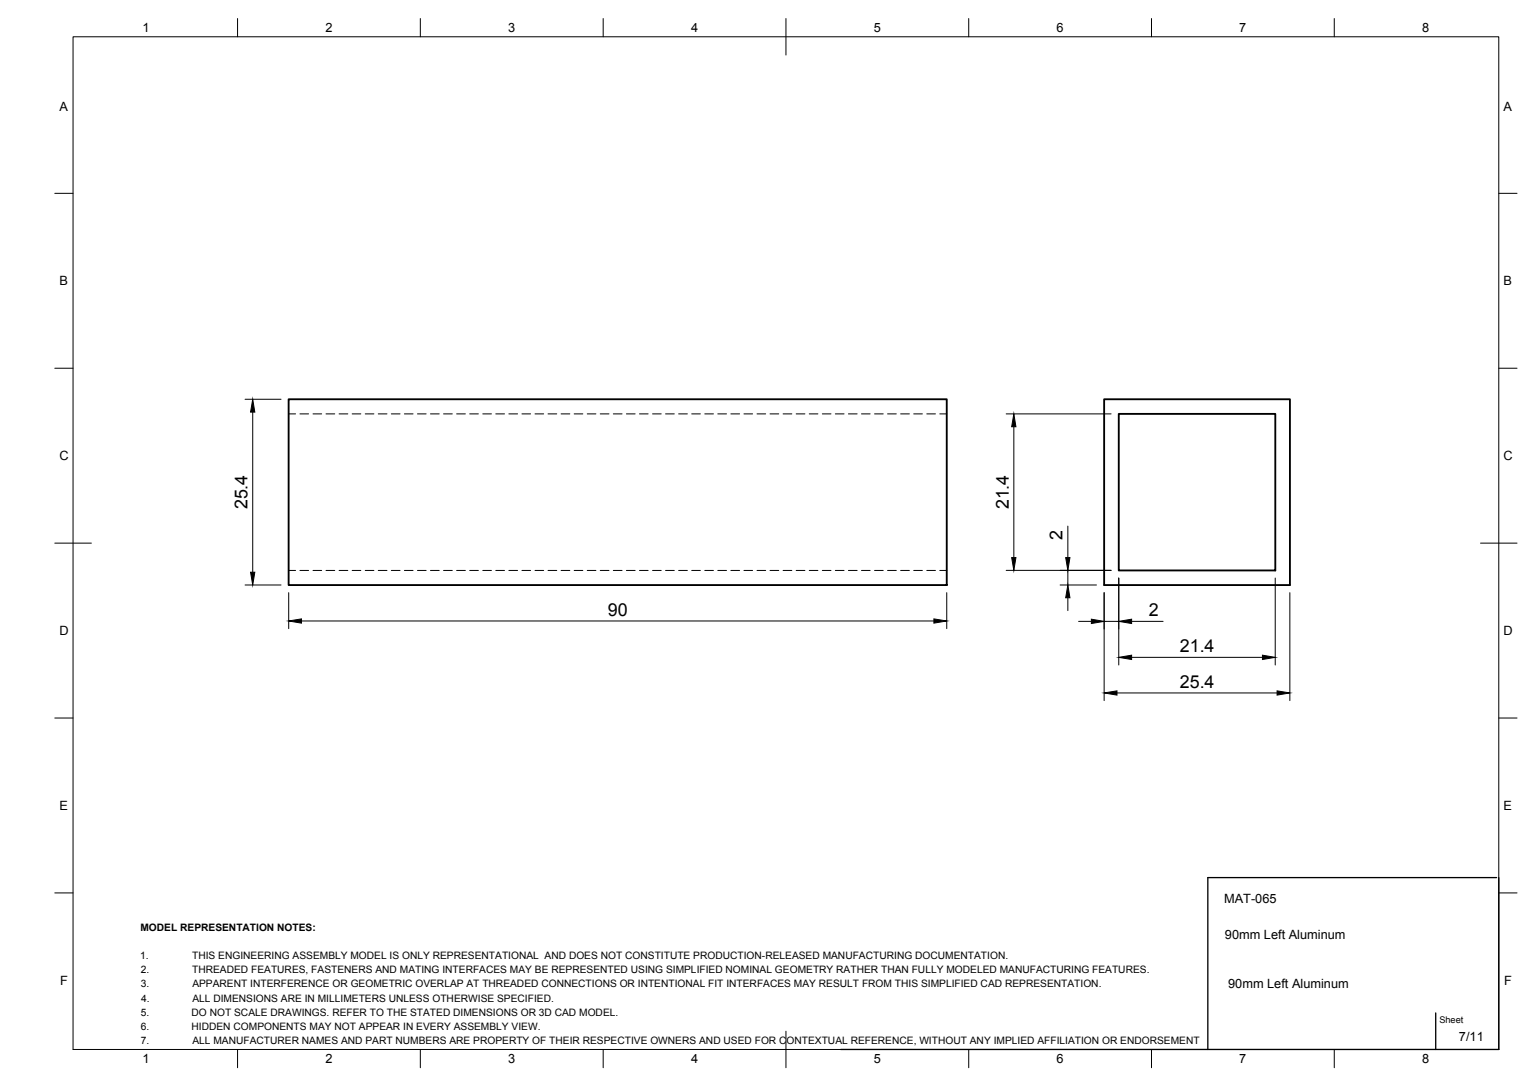
ISO-10303-21;
HEADER;
/* Generated by software containing ST-Developer
 * from STEP Tools, Inc. (www.steptools.com) 
 */

FILE_DESCRIPTION(
/* description */ (
'CAx-IF Rec.Pracs.---Representation and Presentation of Product Manufa
cturing Information (PMI)---4.0---2014-10-13'),
/* implementation_level */ '2;1');

FILE_NAME(
/* name */ '90mm Left Aluminum.step',
/* time_stamp */ '2026-11-15T23:28:27-08:00',
/* author */ (''),
/* organization */ (''),
/* preprocessor_version */ 'ST-DEVELOPER v20.2',
/* originating_system */ 'Autodesk Translation Framework v15.17.0.0',
/* authorisation */ '');

FILE_SCHEMA (('AUTOMOTIVE_DESIGN { 1 0 10303 214 3 1 1 }'));
ENDSEC;

DATA;
#10=MECHANICAL_DESIGN_GEOMETRIC_PRESENTATION_REPRESENTATION('',(#190),#7756);
#172=SHAPE_REPRESENTATION_RELATIONSHIP('SRR','None',#7820,#181);
#181=ADVANCED_BREP_SHAPE_REPRESENTATION('',(#199),#7748);
#190=STYLED_ITEM('',(#7874),#199);
#199=MANIFOLD_SOLID_BREP('Body1',#4627);
#390=FACE_BOUND('',#721,.T.);
#391=FACE_BOUND('',#723,.T.);
#467=FACE_OUTER_BOUND('',#712,.T.);
#468=FACE_OUTER_BOUND('',#713,.T.);
#469=FACE_OUTER_BOUND('',#714,.T.);
#470=FACE_OUTER_BOUND('',#715,.T.);
#471=FACE_OUTER_BOUND('',#716,.T.);
#472=FACE_OUTER_BOUND('',#717,.T.);
#473=FACE_OUTER_BOUND('',#718,.T.);
#474=FACE_OUTER_BOUND('',#719,.T.);
#475=FACE_OUTER_BOUND('',#720,.T.);
#476=FACE_OUTER_BOUND('',#722,.T.);
#712=EDGE_LOOP('',(#3071,#3072,#3073,#3074));
#713=EDGE_LOOP('',(#3075,#3076,#3077,#3078));
#714=EDGE_LOOP('',(#3079,#3080,#3081,#3082));
#715=EDGE_LOOP('',(#3083,#3084,#3085,#3086));
#716=EDGE_LOOP('',(#3087,#3088,#3089,#3090));
#717=EDGE_LOOP('',(#3091,#3092,#3093,#3094));
#718=EDGE_LOOP('',(#3095,#3096,#3097,#3098));
#719=EDGE_LOOP('',(#3099,#3100,#3101,#3102));
#720=EDGE_LOOP('',(#3103,#3104,#3105,#3106));
#721=EDGE_LOOP('',(#3107,#3108,#3109,#3110));
#722=EDGE_LOOP('',(#3111,#3112,#3113,#3114));
#723=EDGE_LOOP('',(#3115,#3116,#3117,#3118));
#1021=LINE('',#6505,#1514);
#1022=LINE('',#6507,#1515);
#1023=LINE('',#6509,#1516);
#1024=LINE('',#6510,#1517);
#1025=LINE('',#6513,#1518);
#1026=LINE('',#6515,#1519);
#1027=LINE('',#6516,#1520);
#1028=LINE('',#6519,#1521);
#1029=LINE('',#6521,#1522);
#1030=LINE('',#6522,#1523);
#1031=LINE('',#6526,#1524);
#1032=LINE('',#6528,#1525);
#1033=LINE('',#6530,#1526);
#1034=LINE('',#6531,#1527);
#1035=LINE('',#6534,#1528);
#1036=LINE('',#6536,#1529);
#1037=LINE('',#6537,#1530);
#1038=LINE('',#6540,#1531);
#1039=LINE('',#6542,#1532);
#1040=LINE('',#6543,#1533);
#1041=LINE('',#6545,#1534);
#1042=LINE('',#6546,#1535);
#1043=LINE('',#6548,#1536);
#1044=LINE('',#6549,#1537);
#1514=VECTOR('',#5219,1.);
#1515=VECTOR('',#5220,1.);
#1516=VECTOR('',#5221,1.);
#1517=VECTOR('',#5222,1.);
#1518=VECTOR('',#5225,1.);
#1519=VECTOR('',#5226,1.);
#1520=VECTOR('',#5227,1.);
#1521=VECTOR('',#5230,1.);
#1522=VECTOR('',#5231,1.);
#1523=VECTOR('',#5232,1.);
#1524=VECTOR('',#5235,1.);
#1525=VECTOR('',#5236,1.);
#1526=VECTOR('',#5237,1.);
#1527=VECTOR('',#5238,1.);
#1528=VECTOR('',#5241,1.);
#1529=VECTOR('',#5242,1.);
#1530=VECTOR('',#5243,1.);
#1531=VECTOR('',#5246,1.);
#1532=VECTOR('',#5247,1.);
#1533=VECTOR('',#5248,1.);
#1534=VECTOR('',#5251,1.);
#1535=VECTOR('',#5252,1.);
#1536=VECTOR('',#5255,1.);
#1537=VECTOR('',#5256,1.);
#2004=VERTEX_POINT('',#6503);
#2005=VERTEX_POINT('',#6504);
#2006=VERTEX_POINT('',#6506);
#2007=VERTEX_POINT('',#6508);
#2008=VERTEX_POINT('',#6512);
#2009=VERTEX_POINT('',#6514);
#2010=VERTEX_POINT('',#6518);
#2011=VERTEX_POINT('',#6520);
#2012=VERTEX_POINT('',#6524);
#2013=VERTEX_POINT('',#6525);
#2014=VERTEX_POINT('',#6527);
#2015=VERTEX_POINT('',#6529);
#2016=VERTEX_POINT('',#6533);
#2017=VERTEX_POINT('',#6535);
#2018=VERTEX_POINT('',#6539);
#2019=VERTEX_POINT('',#6541);
#2419=EDGE_CURVE('',#2004,#2005,#1021,.T.);
#2420=EDGE_CURVE('',#2006,#2004,#1022,.T.);
#2421=EDGE_CURVE('',#2006,#2007,#1023,.T.);
#2422=EDGE_CURVE('',#2007,#2005,#1024,.T.);
#2423=EDGE_CURVE('',#2004,#2008,#1025,.T.);
#2424=EDGE_CURVE('',#2009,#2008,#1026,.T.);
#2425=EDGE_CURVE('',#2006,#2009,#1027,.T.);
#2426=EDGE_CURVE('',#2008,#2010,#1028,.T.);
#2427=EDGE_CURVE('',#2011,#2010,#1029,.T.);
#2428=EDGE_CURVE('',#2009,#2011,#1030,.T.);
#2429=EDGE_CURVE('',#2012,#2013,#1031,.T.);
#2430=EDGE_CURVE('',#2014,#2012,#1032,.T.);
#2431=EDGE_CURVE('',#2014,#2015,#1033,.T.);
#2432=EDGE_CURVE('',#2015,#2013,#1034,.T.);
#2433=EDGE_CURVE('',#2012,#2016,#1035,.T.);
#2434=EDGE_CURVE('',#2017,#2016,#1036,.T.);
#2435=EDGE_CURVE('',#2014,#2017,#1037,.T.);
#2436=EDGE_CURVE('',#2016,#2018,#1038,.T.);
#2437=EDGE_CURVE('',#2019,#2018,#1039,.T.);
#2438=EDGE_CURVE('',#2017,#2019,#1040,.T.);
#2439=EDGE_CURVE('',#2013,#2018,#1041,.T.);
#2440=EDGE_CURVE('',#2015,#2019,#1042,.T.);
#2441=EDGE_CURVE('',#2005,#2010,#1043,.T.);
#2442=EDGE_CURVE('',#2007,#2011,#1044,.T.);
#3071=ORIENTED_EDGE('',*,*,#2419,.F.);
#3072=ORIENTED_EDGE('',*,*,#2420,.F.);
#3073=ORIENTED_EDGE('',*,*,#2421,.T.);
#3074=ORIENTED_EDGE('',*,*,#2422,.T.);
#3075=ORIENTED_EDGE('',*,*,#2423,.T.);
#3076=ORIENTED_EDGE('',*,*,#2424,.F.);
#3077=ORIENTED_EDGE('',*,*,#2425,.F.);
#3078=ORIENTED_EDGE('',*,*,#2420,.T.);
#3079=ORIENTED_EDGE('',*,*,#2426,.T.);
#3080=ORIENTED_EDGE('',*,*,#2427,.F.);
#3081=ORIENTED_EDGE('',*,*,#2428,.F.);
#3082=ORIENTED_EDGE('',*,*,#2424,.T.);
#3083=ORIENTED_EDGE('',*,*,#2429,.F.);
#3084=ORIENTED_EDGE('',*,*,#2430,.F.);
#3085=ORIENTED_EDGE('',*,*,#2431,.T.);
#3086=ORIENTED_EDGE('',*,*,#2432,.T.);
#3087=ORIENTED_EDGE('',*,*,#2433,.T.);
#3088=ORIENTED_EDGE('',*,*,#2434,.F.);
#3089=ORIENTED_EDGE('',*,*,#2435,.F.);
#3090=ORIENTED_EDGE('',*,*,#2430,.T.);
#3091=ORIENTED_EDGE('',*,*,#2436,.T.);
#3092=ORIENTED_EDGE('',*,*,#2437,.F.);
#3093=ORIENTED_EDGE('',*,*,#2438,.F.);
#3094=ORIENTED_EDGE('',*,*,#2434,.T.);
#3095=ORIENTED_EDGE('',*,*,#2439,.F.);
#3096=ORIENTED_EDGE('',*,*,#2432,.F.);
#3097=ORIENTED_EDGE('',*,*,#2440,.T.);
#3098=ORIENTED_EDGE('',*,*,#2437,.T.);
#3099=ORIENTED_EDGE('',*,*,#2441,.F.);
#3100=ORIENTED_EDGE('',*,*,#2422,.F.);
#3101=ORIENTED_EDGE('',*,*,#2442,.T.);
#3102=ORIENTED_EDGE('',*,*,#2427,.T.);
#3103=ORIENTED_EDGE('',*,*,#2421,.F.);
#3104=ORIENTED_EDGE('',*,*,#2425,.T.);
#3105=ORIENTED_EDGE('',*,*,#2428,.T.);
#3106=ORIENTED_EDGE('',*,*,#2442,.F.);
#3107=ORIENTED_EDGE('',*,*,#2431,.F.);
#3108=ORIENTED_EDGE('',*,*,#2435,.T.);
#3109=ORIENTED_EDGE('',*,*,#2438,.T.);
#3110=ORIENTED_EDGE('',*,*,#2440,.F.);
#3111=ORIENTED_EDGE('',*,*,#2419,.T.);
#3112=ORIENTED_EDGE('',*,*,#2441,.T.);
#3113=ORIENTED_EDGE('',*,*,#2426,.F.);
#3114=ORIENTED_EDGE('',*,*,#2423,.F.);
#3115=ORIENTED_EDGE('',*,*,#2429,.T.);
#3116=ORIENTED_EDGE('',*,*,#2439,.T.);
#3117=ORIENTED_EDGE('',*,*,#2436,.F.);
#3118=ORIENTED_EDGE('',*,*,#2433,.F.);
#4229=PLANE('',#4763);
#4230=PLANE('',#4764);
#4231=PLANE('',#4765);
#4232=PLANE('',#4766);
#4233=PLANE('',#4767);
#4234=PLANE('',#4768);
#4235=PLANE('',#4769);
#4236=PLANE('',#4770);
#4237=PLANE('',#4771);
#4238=PLANE('',#4772);
#4408=ADVANCED_FACE('',(#467),#4229,.T.);
#4409=ADVANCED_FACE('',(#468),#4230,.F.);
#4410=ADVANCED_FACE('',(#469),#4231,.F.);
#4411=ADVANCED_FACE('',(#470),#4232,.T.);
#4412=ADVANCED_FACE('',(#471),#4233,.F.);
#4413=ADVANCED_FACE('',(#472),#4234,.F.);
#4414=ADVANCED_FACE('',(#473),#4235,.T.);
#4415=ADVANCED_FACE('',(#474),#4236,.T.);
#4416=ADVANCED_FACE('',(#475,#390),#4237,.T.);
#4417=ADVANCED_FACE('',(#476,#391),#4238,.F.);
#4627=CLOSED_SHELL('',(#4408,#4409,#4410,#4411,#4412,#4413,#4414,#4415,
#4416,#4417));
#4762=AXIS2_PLACEMENT_3D('',#6501,#5215,#5216);
#4763=AXIS2_PLACEMENT_3D('',#6502,#5217,#5218);
#4764=AXIS2_PLACEMENT_3D('',#6511,#5223,#5224);
#4765=AXIS2_PLACEMENT_3D('',#6517,#5228,#5229);
#4766=AXIS2_PLACEMENT_3D('',#6523,#5233,#5234);
#4767=AXIS2_PLACEMENT_3D('',#6532,#5239,#5240);
#4768=AXIS2_PLACEMENT_3D('',#6538,#5244,#5245);
#4769=AXIS2_PLACEMENT_3D('',#6544,#5249,#5250);
#4770=AXIS2_PLACEMENT_3D('',#6547,#5253,#5254);
#4771=AXIS2_PLACEMENT_3D('',#6550,#5257,#5258);
#4772=AXIS2_PLACEMENT_3D('',#6551,#5259,#5260);
#5215=DIRECTION('axis',(0.,0.,1.));
#5216=DIRECTION('refdir',(1.,0.,0.));
#5217=DIRECTION('center_axis',(0.,1.,0.));
#5218=DIRECTION('ref_axis',(0.,0.,1.));
#5219=DIRECTION('',(1.,0.,0.));
#5220=DIRECTION('',(0.,0.,-1.));
#5221=DIRECTION('',(1.,0.,0.));
#5222=DIRECTION('',(0.,0.,-1.));
#5223=DIRECTION('center_axis',(1.,0.,0.));
#5224=DIRECTION('ref_axis',(0.,0.,-1.));
#5225=DIRECTION('',(0.,-1.,0.));
#5226=DIRECTION('',(0.,0.,-1.));
#5227=DIRECTION('',(0.,-1.,0.));
#5228=DIRECTION('center_axis',(0.,1.,0.));
#5229=DIRECTION('ref_axis',(0.,0.,1.));
#5230=DIRECTION('',(1.,0.,0.));
#5231=DIRECTION('',(0.,0.,-1.));
#5232=DIRECTION('',(1.,0.,0.));
#5233=DIRECTION('center_axis',(1.,0.,0.));
#5234=DIRECTION('ref_axis',(0.,0.,-1.));
#5235=DIRECTION('',(0.,-1.,0.));
#5236=DIRECTION('',(0.,0.,-1.));
#5237=DIRECTION('',(0.,-1.,0.));
#5238=DIRECTION('',(0.,0.,-1.));
#5239=DIRECTION('center_axis',(0.,1.,0.));
#5240=DIRECTION('ref_axis',(0.,0.,1.));
#5241=DIRECTION('',(1.,0.,0.));
#5242=DIRECTION('',(0.,0.,-1.));
#5243=DIRECTION('',(1.,0.,0.));
#5244=DIRECTION('center_axis',(1.,0.,0.));
#5245=DIRECTION('ref_axis',(0.,0.,-1.));
#5246=DIRECTION('',(0.,-1.,0.));
#5247=DIRECTION('',(0.,0.,-1.));
#5248=DIRECTION('',(0.,-1.,0.));
#5249=DIRECTION('center_axis',(0.,1.,0.));
#5250=DIRECTION('ref_axis',(0.,0.,1.));
#5251=DIRECTION('',(1.,0.,0.));
#5252=DIRECTION('',(1.,0.,0.));
#5253=DIRECTION('center_axis',(1.,0.,0.));
#5254=DIRECTION('ref_axis',(0.,0.,-1.));
#5255=DIRECTION('',(0.,-1.,0.));
#5256=DIRECTION('',(0.,-1.,0.));
#5257=DIRECTION('center_axis',(0.,0.,1.));
#5258=DIRECTION('ref_axis',(1.,0.,0.));
#5259=DIRECTION('center_axis',(0.,0.,1.));
#5260=DIRECTION('ref_axis',(1.,0.,0.));
#6501=CARTESIAN_POINT('',(0.,0.,0.));
#6502=CARTESIAN_POINT('Origin',(0.0208455896936357,0.0585086531437975,0.09));
#6503=CARTESIAN_POINT('',(0.0081455896936357,0.0585086531437975,0.));
#6504=CARTESIAN_POINT('',(0.0335455896936357,0.0585086531437975,0.));
#6505=CARTESIAN_POINT('',(0.0208455896936357,0.0585086531437975,0.));
#6506=CARTESIAN_POINT('',(0.0081455896936357,0.0585086531437975,0.09));
#6507=CARTESIAN_POINT('',(0.0081455896936357,0.0585086531437975,0.09));
#6508=CARTESIAN_POINT('',(0.0335455896936357,0.0585086531437975,0.09));
#6509=CARTESIAN_POINT('',(0.0208455896936357,0.0585086531437975,0.09));
#6510=CARTESIAN_POINT('',(0.0335455896936357,0.0585086531437975,0.09));
#6511=CARTESIAN_POINT('Origin',(0.0081455896936357,0.0458086531437975,0.09));
#6512=CARTESIAN_POINT('',(0.0081455896936357,0.0331086531437976,0.));
#6513=CARTESIAN_POINT('',(0.0081455896936357,0.0458086531437975,0.));
#6514=CARTESIAN_POINT('',(0.0081455896936357,0.0331086531437976,0.09));
#6515=CARTESIAN_POINT('',(0.0081455896936357,0.0331086531437976,0.09));
#6516=CARTESIAN_POINT('',(0.0081455896936357,0.0458086531437975,0.09));
#6517=CARTESIAN_POINT('Origin',(0.0208455896936357,0.0331086531437976,0.09));
#6518=CARTESIAN_POINT('',(0.0335455896936357,0.0331086531437976,0.));
#6519=CARTESIAN_POINT('',(0.0208455896936357,0.0331086531437976,0.));
#6520=CARTESIAN_POINT('',(0.0335455896936357,0.0331086531437976,0.09));
#6521=CARTESIAN_POINT('',(0.0335455896936357,0.0331086531437976,0.09));
#6522=CARTESIAN_POINT('',(0.0208455896936357,0.0331086531437976,0.09));
#6523=CARTESIAN_POINT('Origin',(0.0101455896936357,0.0458086531437976,0.09));
#6524=CARTESIAN_POINT('',(0.0101455896936357,0.0565086531437975,0.));
#6525=CARTESIAN_POINT('',(0.0101455896936357,0.0351086531437975,0.));
#6526=CARTESIAN_POINT('',(0.0101455896936357,0.0458086531437976,0.));
#6527=CARTESIAN_POINT('',(0.0101455896936357,0.0565086531437975,0.09));
#6528=CARTESIAN_POINT('',(0.0101455896936357,0.0565086531437975,0.09));
#6529=CARTESIAN_POINT('',(0.0101455896936357,0.0351086531437975,0.09));
#6530=CARTESIAN_POINT('',(0.0101455896936357,0.0458086531437976,0.09));
#6531=CARTESIAN_POINT('',(0.0101455896936357,0.0351086531437975,0.09));
#6532=CARTESIAN_POINT('Origin',(0.0208455896936357,0.0565086531437975,0.09));
#6533=CARTESIAN_POINT('',(0.0315455896936357,0.0565086531437975,0.));
#6534=CARTESIAN_POINT('',(0.0208455896936357,0.0565086531437975,0.));
#6535=CARTESIAN_POINT('',(0.0315455896936357,0.0565086531437975,0.09));
#6536=CARTESIAN_POINT('',(0.0315455896936357,0.0565086531437975,0.09));
#6537=CARTESIAN_POINT('',(0.0208455896936357,0.0565086531437975,0.09));
#6538=CARTESIAN_POINT('Origin',(0.0315455896936357,0.0458086531437976,0.09));
#6539=CARTESIAN_POINT('',(0.0315455896936357,0.0351086531437975,0.));
#6540=CARTESIAN_POINT('',(0.0315455896936357,0.0458086531437976,0.));
#6541=CARTESIAN_POINT('',(0.0315455896936357,0.0351086531437975,0.09));
#6542=CARTESIAN_POINT('',(0.0315455896936357,0.0351086531437975,0.09));
#6543=CARTESIAN_POINT('',(0.0315455896936357,0.0458086531437976,0.09));
#6544=CARTESIAN_POINT('Origin',(0.0208455896936357,0.0351086531437975,0.09));
#6545=CARTESIAN_POINT('',(0.0208455896936357,0.0351086531437975,0.));
#6546=CARTESIAN_POINT('',(0.0208455896936357,0.0351086531437975,0.09));
#6547=CARTESIAN_POINT('Origin',(0.0335455896936357,0.0458086531437975,0.09));
#6548=CARTESIAN_POINT('',(0.0335455896936357,0.0458086531437975,0.));
#6549=CARTESIAN_POINT('',(0.0335455896936357,0.0458086531437975,0.09));
#6550=CARTESIAN_POINT('Origin',(0.0208455896936357,0.0458086531437975,0.09));
#6551=CARTESIAN_POINT('Origin',(0.0208455896936357,0.0458086531437975,0.));
#7737=UNCERTAINTY_MEASURE_WITH_UNIT(LENGTH_MEASURE(1.E-5),#7757,
'DISTANCE_ACCURACY_VALUE',
'Maximum model space distance between geometric entities at asserted c
onnectivities');
#7745=UNCERTAINTY_MEASURE_WITH_UNIT(LENGTH_MEASURE(1.E-5),#7757,
'DISTANCE_ACCURACY_VALUE',
'Maximum model space distance between geometric entities at asserted c
onnectivities');
#7748=(
GEOMETRIC_REPRESENTATION_CONTEXT(3)
GLOBAL_UNCERTAINTY_ASSIGNED_CONTEXT((#7737))
GLOBAL_UNIT_ASSIGNED_CONTEXT((#7757,#7758,#7759))
REPRESENTATION_CONTEXT('','3D')
);
#7756=(
GEOMETRIC_REPRESENTATION_CONTEXT(3)
GLOBAL_UNCERTAINTY_ASSIGNED_CONTEXT((#7745))
GLOBAL_UNIT_ASSIGNED_CONTEXT((#7757,#7758,#7759))
REPRESENTATION_CONTEXT('','3D')
);
#7757=(
LENGTH_UNIT()
NAMED_UNIT(*)
SI_UNIT($,.METRE.)
);
#7758=(
NAMED_UNIT(*)
PLANE_ANGLE_UNIT()
SI_UNIT($,.RADIAN.)
);
#7759=(
NAMED_UNIT(*)
SI_UNIT($,.STERADIAN.)
SOLID_ANGLE_UNIT()
);
#7762=SHAPE_DEFINITION_REPRESENTATION(#7772,#7820);
#7772=PRODUCT_DEFINITION_SHAPE('',$,#7831);
#7820=SHAPE_REPRESENTATION('',(#4762),#7748);
#7828=PRODUCT_DEFINITION_CONTEXT('part definition',#7860,'design');
#7831=PRODUCT_DEFINITION('90mm Left Aluminum','90mm Left Aluminum',#7841,
#7828);
#7841=PRODUCT_DEFINITION_FORMATION('',$,#7864);
#7860=APPLICATION_CONTEXT(
'Core Data for Automotive Mechanical Design Process');
#7861=PRODUCT_CONTEXT('part definition',#7860,'mechanical');
#7864=PRODUCT('90mm Left Aluminum','90mm Left Aluminum',
'LEGAL AND USAGE DISCLAIMER: this Data/Model is provided \X2\201C\X0\A
S IS\X2\201D\X0\ for informational and representational only. It is a 
geometric approximation and is NOT engineered, certified, or guarantee
d for dimensional accuracy, exact tolerances, or production-level prec
ision. Vendor disclaims all implied warranties including fitness for a
 particular purpose. DO NOT USE FOR DIRECT PHYSICAL MANUFACTURING, AUT
OMATED PRODUCTION, OR SAFETY-CRITICAL SYSTEMS without independent engi
neering verification and resolution of any design discrepancies.',(#7861));
#7874=PRESENTATION_STYLE_ASSIGNMENT((#7881));
#7881=SURFACE_STYLE_USAGE(.BOTH.,#7888);
#7888=SURFACE_SIDE_STYLE('',(#7895));
#7895=SURFACE_STYLE_FILL_AREA(#7902);
#7902=FILL_AREA_STYLE('Opaque(179,179,179)',(#7909));
#7909=FILL_AREA_STYLE_COLOUR('Opaque(179,179,179)',#7916);
#7916=COLOUR_RGB('Opaque(179,179,179)',0.701960784313725,0.701960784313725,
0.701960784313725);
ENDSEC;
END-ISO-10303-21;
